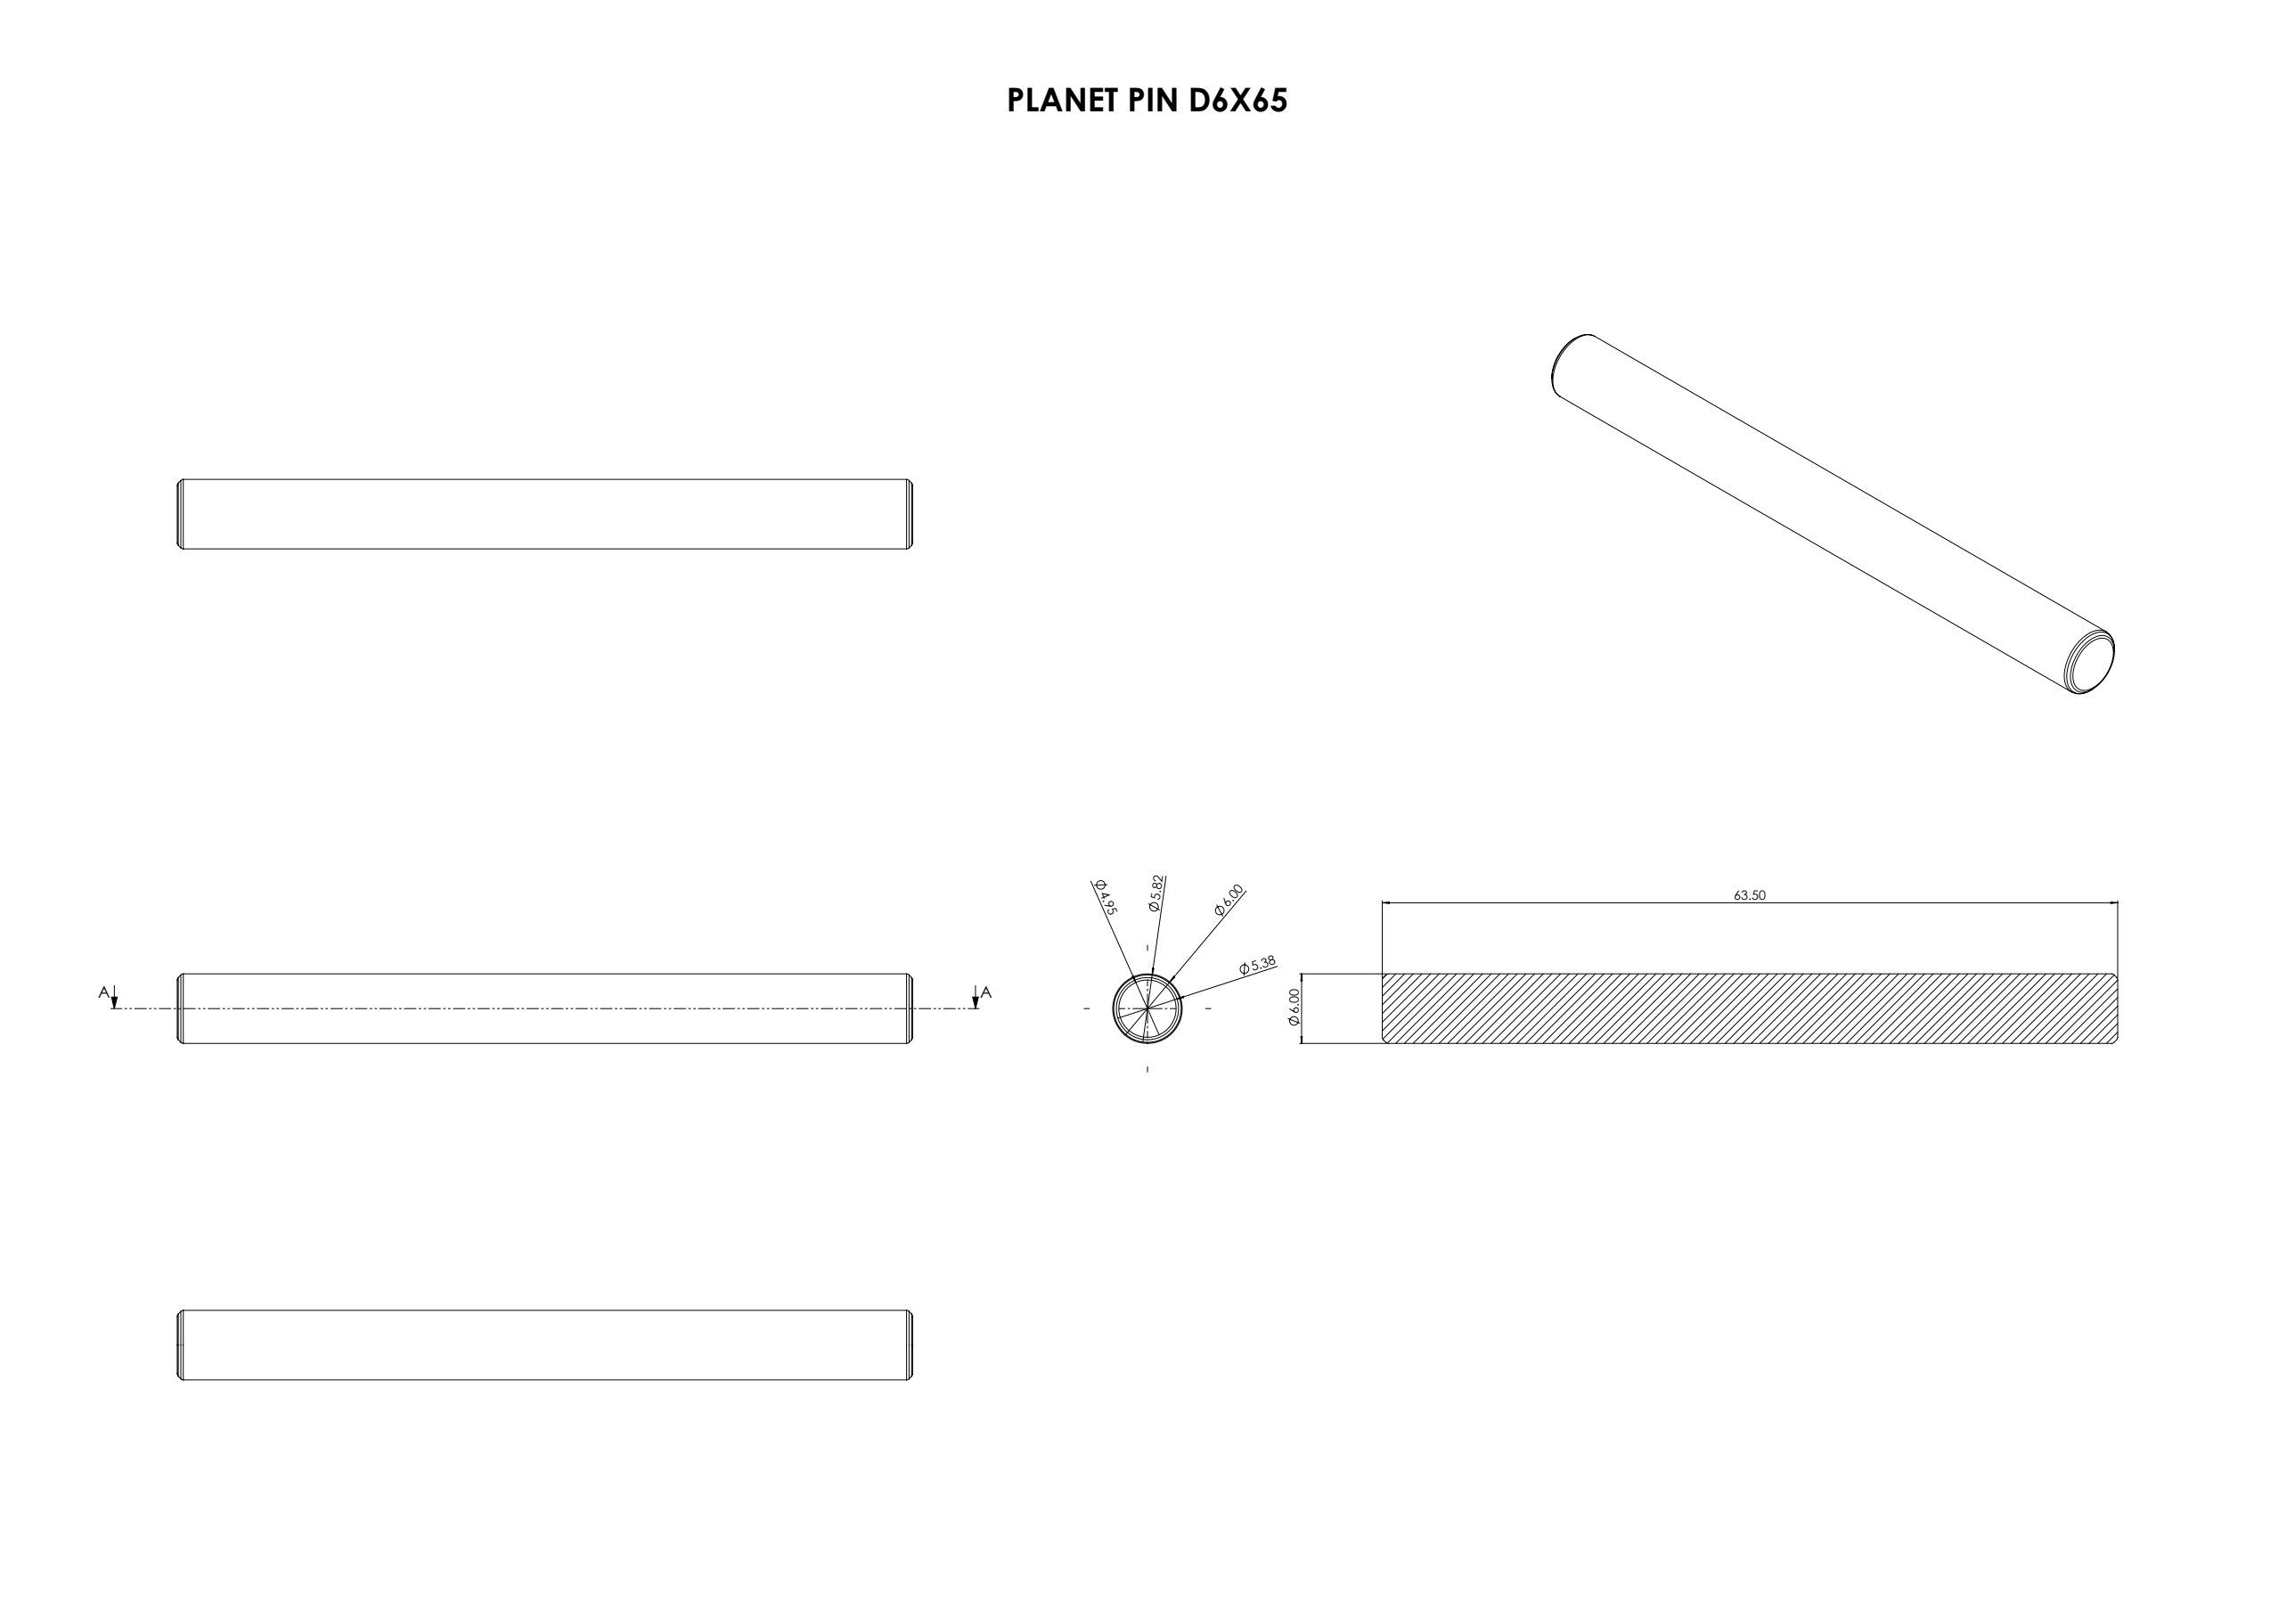
ISO-10303-21;
HEADER;
/* Generated by software containing ST-Developer
 * from STEP Tools, Inc. (www.steptools.com) 
 */

FILE_DESCRIPTION(
/* description */ (''),
/* implementation_level */ '2;1');

FILE_NAME(
/* name */ '04_Planet_Pin_D6x65.step',
/* time_stamp */ '2026-10-11T13:00:10-07:00',
/* author */ (''),
/* organization */ (''),
/* preprocessor_version */ 'ST-DEVELOPER v20.2',
/* originating_system */ 'Autodesk Translation Framework v15.15.0.0',
/* authorisation */ '');

FILE_SCHEMA (('AUTOMOTIVE_DESIGN { 1 0 10303 214 3 1 1 }'));
ENDSEC;

DATA;
#10=MECHANICAL_DESIGN_GEOMETRIC_PRESENTATION_REPRESENTATION('',(#361),#65563);
#145=TOROIDAL_SURFACE('',#21674,2.47573593128807,0.3);
#146=TOROIDAL_SURFACE('',#21683,2.7,0.3);
#147=TOROIDAL_SURFACE('',#21690,2.7,0.3);
#148=TOROIDAL_SURFACE('',#21697,2.47573593128807,0.3);
#339=SHAPE_REPRESENTATION_RELATIONSHIP('SRR','None',#65617,#350);
#350=ADVANCED_BREP_SHAPE_REPRESENTATION('',(#372),#65555);
#361=STYLED_ITEM('',(#65788),#372);
#372=MANIFOLD_SOLID_BREP('Body1',#20011);
#489=CONICAL_SURFACE('',#21679,2.8,0.785398163397448);
#490=CONICAL_SURFACE('',#21694,2.8,0.785398163397436);
#974=PLANE('',#21682);
#975=PLANE('',#21700);
#1978=FACE_OUTER_BOUND('',#3200,.T.);
#1979=FACE_OUTER_BOUND('',#3201,.T.);
#1980=FACE_OUTER_BOUND('',#3202,.T.);
#1981=FACE_OUTER_BOUND('',#3203,.T.);
#1982=FACE_OUTER_BOUND('',#3204,.T.);
#1983=FACE_OUTER_BOUND('',#3205,.T.);
#1984=FACE_OUTER_BOUND('',#3206,.T.);
#1985=FACE_OUTER_BOUND('',#3207,.T.);
#1986=FACE_OUTER_BOUND('',#3208,.T.);
#3200=EDGE_LOOP('',(#16702,#16703,#16704,#16705,#16706));
#3201=EDGE_LOOP('',(#16707,#16708,#16709,#16710,#16711,#16712));
#3202=EDGE_LOOP('',(#16713));
#3203=EDGE_LOOP('',(#16714,#16715,#16716,#16717,#16718,#16719));
#3204=EDGE_LOOP('',(#16720,#16721,#16722,#16723,#16724,#16725));
#3205=EDGE_LOOP('',(#16726,#16727,#16728,#16729,#16730,#16731));
#3206=EDGE_LOOP('',(#16732,#16733,#16734,#16735,#16736,#16737));
#3207=EDGE_LOOP('',(#16738,#16739,#16740,#16741,#16742));
#3208=EDGE_LOOP('',(#16743));
#4302=CIRCLE('',#21675,2.47573593128807);
#4303=CIRCLE('',#21676,0.3);
#4304=CIRCLE('',#21677,2.68786796564404);
#4305=CIRCLE('',#21678,2.68786796564404);
#4306=CIRCLE('',#21680,2.91213203435596);
#4307=CIRCLE('',#21681,2.91213203435596);
#4308=CIRCLE('',#21684,0.3);
#4309=CIRCLE('',#21685,3.);
#4310=CIRCLE('',#21686,3.);
#4311=CIRCLE('',#21688,3.);
#4312=CIRCLE('',#21689,3.);
#4313=CIRCLE('',#21691,0.3);
#4314=CIRCLE('',#21692,2.91213203435597);
#4315=CIRCLE('',#21693,2.91213203435597);
#4316=CIRCLE('',#21695,2.68786796564404);
#4317=CIRCLE('',#21696,2.68786796564404);
#4318=CIRCLE('',#21698,0.3);
#4319=CIRCLE('',#21699,2.47573593128807);
#6007=LINE('',#61837,#6899);
#6008=LINE('',#61850,#6900);
#6009=LINE('',#61862,#6901);
#6899=VECTOR('',#26046,2.8);
#6900=VECTOR('',#26063,3.);
#6901=VECTOR('',#26078,2.8);
#8647=VERTEX_POINT('',#61828);
#8648=VERTEX_POINT('',#61830);
#8649=VERTEX_POINT('',#61832);
#8650=VERTEX_POINT('',#61836);
#8651=VERTEX_POINT('',#61838);
#8652=VERTEX_POINT('',#61843);
#8653=VERTEX_POINT('',#61845);
#8654=VERTEX_POINT('',#61849);
#8655=VERTEX_POINT('',#61851);
#8656=VERTEX_POINT('',#61855);
#8657=VERTEX_POINT('',#61857);
#8658=VERTEX_POINT('',#61861);
#8659=VERTEX_POINT('',#61863);
#8660=VERTEX_POINT('',#61867);
#11384=EDGE_CURVE('',#8647,#8647,#4302,.T.);
#11385=EDGE_CURVE('',#8647,#8648,#4303,.T.);
#11386=EDGE_CURVE('',#8648,#8649,#4304,.T.);
#11387=EDGE_CURVE('',#8649,#8648,#4305,.T.);
#11388=EDGE_CURVE('',#8649,#8650,#6007,.T.);
#11389=EDGE_CURVE('',#8651,#8650,#4306,.T.);
#11390=EDGE_CURVE('',#8650,#8651,#4307,.T.);
#11391=EDGE_CURVE('',#8651,#8652,#4308,.T.);
#11392=EDGE_CURVE('',#8652,#8653,#4309,.T.);
#11393=EDGE_CURVE('',#8653,#8652,#4310,.T.);
#11394=EDGE_CURVE('',#8653,#8654,#6008,.T.);
#11395=EDGE_CURVE('',#8655,#8654,#4311,.T.);
#11396=EDGE_CURVE('',#8654,#8655,#4312,.T.);
#11397=EDGE_CURVE('',#8655,#8656,#4313,.T.);
#11398=EDGE_CURVE('',#8656,#8657,#4314,.T.);
#11399=EDGE_CURVE('',#8657,#8656,#4315,.T.);
#11400=EDGE_CURVE('',#8657,#8658,#6009,.T.);
#11401=EDGE_CURVE('',#8659,#8658,#4316,.T.);
#11402=EDGE_CURVE('',#8658,#8659,#4317,.T.);
#11403=EDGE_CURVE('',#8659,#8660,#4318,.T.);
#11404=EDGE_CURVE('',#8660,#8660,#4319,.T.);
#16702=ORIENTED_EDGE('',*,*,#11384,.T.);
#16703=ORIENTED_EDGE('',*,*,#11385,.T.);
#16704=ORIENTED_EDGE('',*,*,#11386,.T.);
#16705=ORIENTED_EDGE('',*,*,#11387,.T.);
#16706=ORIENTED_EDGE('',*,*,#11385,.F.);
#16707=ORIENTED_EDGE('',*,*,#11387,.F.);
#16708=ORIENTED_EDGE('',*,*,#11388,.T.);
#16709=ORIENTED_EDGE('',*,*,#11389,.F.);
#16710=ORIENTED_EDGE('',*,*,#11390,.F.);
#16711=ORIENTED_EDGE('',*,*,#11388,.F.);
#16712=ORIENTED_EDGE('',*,*,#11386,.F.);
#16713=ORIENTED_EDGE('',*,*,#11384,.F.);
#16714=ORIENTED_EDGE('',*,*,#11389,.T.);
#16715=ORIENTED_EDGE('',*,*,#11390,.T.);
#16716=ORIENTED_EDGE('',*,*,#11391,.T.);
#16717=ORIENTED_EDGE('',*,*,#11392,.T.);
#16718=ORIENTED_EDGE('',*,*,#11393,.T.);
#16719=ORIENTED_EDGE('',*,*,#11391,.F.);
#16720=ORIENTED_EDGE('',*,*,#11393,.F.);
#16721=ORIENTED_EDGE('',*,*,#11394,.T.);
#16722=ORIENTED_EDGE('',*,*,#11395,.F.);
#16723=ORIENTED_EDGE('',*,*,#11396,.F.);
#16724=ORIENTED_EDGE('',*,*,#11394,.F.);
#16725=ORIENTED_EDGE('',*,*,#11392,.F.);
#16726=ORIENTED_EDGE('',*,*,#11395,.T.);
#16727=ORIENTED_EDGE('',*,*,#11396,.T.);
#16728=ORIENTED_EDGE('',*,*,#11397,.T.);
#16729=ORIENTED_EDGE('',*,*,#11398,.T.);
#16730=ORIENTED_EDGE('',*,*,#11399,.T.);
#16731=ORIENTED_EDGE('',*,*,#11397,.F.);
#16732=ORIENTED_EDGE('',*,*,#11399,.F.);
#16733=ORIENTED_EDGE('',*,*,#11400,.T.);
#16734=ORIENTED_EDGE('',*,*,#11401,.F.);
#16735=ORIENTED_EDGE('',*,*,#11402,.F.);
#16736=ORIENTED_EDGE('',*,*,#11400,.F.);
#16737=ORIENTED_EDGE('',*,*,#11398,.F.);
#16738=ORIENTED_EDGE('',*,*,#11401,.T.);
#16739=ORIENTED_EDGE('',*,*,#11402,.T.);
#16740=ORIENTED_EDGE('',*,*,#11403,.T.);
#16741=ORIENTED_EDGE('',*,*,#11404,.T.);
#16742=ORIENTED_EDGE('',*,*,#11403,.F.);
#16743=ORIENTED_EDGE('',*,*,#11404,.F.);
#18716=CYLINDRICAL_SURFACE('',#21687,3.);
#19674=ADVANCED_FACE('',(#1978),#145,.T.);
#19675=ADVANCED_FACE('',(#1979),#489,.T.);
#19676=ADVANCED_FACE('',(#1980),#974,.T.);
#19677=ADVANCED_FACE('',(#1981),#146,.T.);
#19678=ADVANCED_FACE('',(#1982),#18716,.T.);
#19679=ADVANCED_FACE('',(#1983),#147,.T.);
#19680=ADVANCED_FACE('',(#1984),#490,.T.);
#19681=ADVANCED_FACE('',(#1985),#148,.T.);
#19682=ADVANCED_FACE('',(#1986),#975,.T.);
#20011=CLOSED_SHELL('',(#19674,#19675,#19676,#19677,#19678,#19679,#19680,
#19681,#19682));
#21673=AXIS2_PLACEMENT_3D('',#61826,#26032,#26033);
#21674=AXIS2_PLACEMENT_3D('',#61827,#26034,#26035);
#21675=AXIS2_PLACEMENT_3D('',#61829,#26036,#26037);
#21676=AXIS2_PLACEMENT_3D('',#61831,#26038,#26039);
#21677=AXIS2_PLACEMENT_3D('',#61833,#26040,#26041);
#21678=AXIS2_PLACEMENT_3D('',#61834,#26042,#26043);
#21679=AXIS2_PLACEMENT_3D('',#61835,#26044,#26045);
#21680=AXIS2_PLACEMENT_3D('',#61839,#26047,#26048);
#21681=AXIS2_PLACEMENT_3D('',#61840,#26049,#26050);
#21682=AXIS2_PLACEMENT_3D('',#61841,#26051,#26052);
#21683=AXIS2_PLACEMENT_3D('',#61842,#26053,#26054);
#21684=AXIS2_PLACEMENT_3D('',#61844,#26055,#26056);
#21685=AXIS2_PLACEMENT_3D('',#61846,#26057,#26058);
#21686=AXIS2_PLACEMENT_3D('',#61847,#26059,#26060);
#21687=AXIS2_PLACEMENT_3D('',#61848,#26061,#26062);
#21688=AXIS2_PLACEMENT_3D('',#61852,#26064,#26065);
#21689=AXIS2_PLACEMENT_3D('',#61853,#26066,#26067);
#21690=AXIS2_PLACEMENT_3D('',#61854,#26068,#26069);
#21691=AXIS2_PLACEMENT_3D('',#61856,#26070,#26071);
#21692=AXIS2_PLACEMENT_3D('',#61858,#26072,#26073);
#21693=AXIS2_PLACEMENT_3D('',#61859,#26074,#26075);
#21694=AXIS2_PLACEMENT_3D('',#61860,#26076,#26077);
#21695=AXIS2_PLACEMENT_3D('',#61864,#26079,#26080);
#21696=AXIS2_PLACEMENT_3D('',#61865,#26081,#26082);
#21697=AXIS2_PLACEMENT_3D('',#61866,#26083,#26084);
#21698=AXIS2_PLACEMENT_3D('',#61868,#26085,#26086);
#21699=AXIS2_PLACEMENT_3D('',#61869,#26087,#26088);
#21700=AXIS2_PLACEMENT_3D('',#61870,#26089,#26090);
#26032=DIRECTION('axis',(0.,0.,1.));
#26033=DIRECTION('refdir',(1.,0.,0.));
#26034=DIRECTION('center_axis',(1.,0.,0.));
#26035=DIRECTION('ref_axis',(0.,0.,-1.));
#26036=DIRECTION('center_axis',(-1.,0.,0.));
#26037=DIRECTION('ref_axis',(0.,-1.,1.83697019872103E-16));
#26038=DIRECTION('center_axis',(0.,-1.,-1.22464679914735E-16));
#26039=DIRECTION('ref_axis',(0.,-1.22464679914735E-16,1.));
#26040=DIRECTION('center_axis',(1.,0.,0.));
#26041=DIRECTION('ref_axis',(0.,-1.,3.06161699786838E-17));
#26042=DIRECTION('center_axis',(1.,0.,0.));
#26043=DIRECTION('ref_axis',(0.,-1.,3.06161699786838E-17));
#26044=DIRECTION('center_axis',(-1.,0.,0.));
#26045=DIRECTION('ref_axis',(0.,1.,0.));
#26046=DIRECTION('',(-0.707106781186548,-0.707106781186547,-8.65956056235493E-17));
#26047=DIRECTION('center_axis',(-1.,0.,0.));
#26048=DIRECTION('ref_axis',(0.,-1.,3.06161699786838E-17));
#26049=DIRECTION('center_axis',(-1.,0.,0.));
#26050=DIRECTION('ref_axis',(0.,-1.,3.06161699786838E-17));
#26051=DIRECTION('center_axis',(1.,0.,0.));
#26052=DIRECTION('ref_axis',(0.,0.,-1.));
#26053=DIRECTION('center_axis',(1.,0.,0.));
#26054=DIRECTION('ref_axis',(0.,0.,-1.));
#26055=DIRECTION('center_axis',(0.,-1.,-1.22464679914735E-16));
#26056=DIRECTION('ref_axis',(0.,-1.22464679914735E-16,1.));
#26057=DIRECTION('center_axis',(1.,0.,0.));
#26058=DIRECTION('ref_axis',(0.,-1.,1.83697019872103E-16));
#26059=DIRECTION('center_axis',(1.,0.,0.));
#26060=DIRECTION('ref_axis',(0.,-1.,1.83697019872103E-16));
#26061=DIRECTION('center_axis',(1.,0.,0.));
#26062=DIRECTION('ref_axis',(0.,1.,0.));
#26063=DIRECTION('',(-1.,0.,0.));
#26064=DIRECTION('center_axis',(-1.,0.,0.));
#26065=DIRECTION('ref_axis',(0.,-1.,1.83697019872103E-16));
#26066=DIRECTION('center_axis',(-1.,0.,0.));
#26067=DIRECTION('ref_axis',(0.,-1.,1.83697019872103E-16));
#26068=DIRECTION('center_axis',(1.,0.,0.));
#26069=DIRECTION('ref_axis',(0.,0.,-1.));
#26070=DIRECTION('center_axis',(0.,-1.,-1.22464679914735E-16));
#26071=DIRECTION('ref_axis',(0.,-1.22464679914735E-16,1.));
#26072=DIRECTION('center_axis',(1.,0.,0.));
#26073=DIRECTION('ref_axis',(0.,-1.,3.06161699786838E-17));
#26074=DIRECTION('center_axis',(1.,0.,0.));
#26075=DIRECTION('ref_axis',(0.,-1.,3.06161699786838E-17));
#26076=DIRECTION('center_axis',(1.,0.,0.));
#26077=DIRECTION('ref_axis',(0.,1.,0.));
#26078=DIRECTION('',(-0.707106781186556,0.707106781186539,8.65956056235483E-17));
#26079=DIRECTION('center_axis',(-1.,0.,0.));
#26080=DIRECTION('ref_axis',(0.,-1.,3.06161699786838E-17));
#26081=DIRECTION('center_axis',(-1.,0.,0.));
#26082=DIRECTION('ref_axis',(0.,-1.,3.06161699786838E-17));
#26083=DIRECTION('center_axis',(1.,0.,0.));
#26084=DIRECTION('ref_axis',(0.,0.,-1.));
#26085=DIRECTION('center_axis',(0.,-1.,-1.22464679914735E-16));
#26086=DIRECTION('ref_axis',(0.,-1.22464679914735E-16,1.));
#26087=DIRECTION('center_axis',(1.,0.,0.));
#26088=DIRECTION('ref_axis',(0.,-1.,1.83697019872103E-16));
#26089=DIRECTION('center_axis',(-1.,0.,0.));
#26090=DIRECTION('ref_axis',(0.,0.,1.));
#61826=CARTESIAN_POINT('',(0.,0.,0.));
#61827=CARTESIAN_POINT('Origin',(-15.8,0.,0.));
#61828=CARTESIAN_POINT('',(-15.5,-3.03190208378603E-16,2.47573593128807));
#61829=CARTESIAN_POINT('Origin',(-15.5,0.,0.));
#61830=CARTESIAN_POINT('',(-15.587867965644,-3.29168890065668E-16,2.68786796564404));
#61831=CARTESIAN_POINT('Origin',(-15.8,-3.03190208378603E-16,2.47573593128807));
#61832=CARTESIAN_POINT('',(-15.587867965644,-2.68786796564404,-3.29168890065668E-16));
#61833=CARTESIAN_POINT('Origin',(-15.587867965644,0.,-4.11461112582085E-16));
#61834=CARTESIAN_POINT('Origin',(-15.587867965644,0.,-4.11461112582085E-16));
#61835=CARTESIAN_POINT('Origin',(-15.7,0.,0.));
#61836=CARTESIAN_POINT('',(-15.812132034356,-2.91213203435596,-3.5663331745685E-16));
#61837=CARTESIAN_POINT('',(-15.7,-2.8,-3.42901103761259E-16));
#61838=CARTESIAN_POINT('',(-15.812132034356,-3.5663331745685E-16,2.91213203435596));
#61839=CARTESIAN_POINT('Origin',(-15.812132034356,0.,-4.45791646821063E-16));
#61840=CARTESIAN_POINT('Origin',(-15.812132034356,0.,-4.45791646821063E-16));
#61841=CARTESIAN_POINT('Origin',(-15.5,0.,0.));
#61842=CARTESIAN_POINT('Origin',(-16.0242640687119,0.,0.));
#61843=CARTESIAN_POINT('',(-16.0242640687119,-3.67394039744206E-16,3.));
#61844=CARTESIAN_POINT('Origin',(-16.0242640687119,-3.30654635769785E-16,
2.7));
#61845=CARTESIAN_POINT('',(-16.0242640687119,-3.,-3.67394039744206E-16));
#61846=CARTESIAN_POINT('Origin',(-16.0242640687119,0.,0.));
#61847=CARTESIAN_POINT('Origin',(-16.0242640687119,0.,0.));
#61848=CARTESIAN_POINT('Origin',(-47.25,0.,0.));
#61849=CARTESIAN_POINT('',(-78.4757359312881,-3.,-3.67394039744206E-16));
#61850=CARTESIAN_POINT('',(-47.25,-3.,-3.67394039744206E-16));
#61851=CARTESIAN_POINT('',(-78.4757359312881,-3.67394039744206E-16,3.));
#61852=CARTESIAN_POINT('Origin',(-78.4757359312881,0.,0.));
#61853=CARTESIAN_POINT('Origin',(-78.4757359312881,0.,0.));
#61854=CARTESIAN_POINT('Origin',(-78.4757359312881,0.,0.));
#61855=CARTESIAN_POINT('',(-78.687867965644,-3.5663331745685E-16,2.91213203435596));
#61856=CARTESIAN_POINT('Origin',(-78.4757359312881,-3.30654635769785E-16,
2.7));
#61857=CARTESIAN_POINT('',(-78.687867965644,-2.91213203435597,-3.5663331745685E-16));
#61858=CARTESIAN_POINT('Origin',(-78.687867965644,0.,-4.45791646821063E-16));
#61859=CARTESIAN_POINT('Origin',(-78.687867965644,0.,-4.45791646821063E-16));
#61860=CARTESIAN_POINT('Origin',(-78.8,0.,0.));
#61861=CARTESIAN_POINT('',(-78.912132034356,-2.68786796564404,-3.29168890065668E-16));
#61862=CARTESIAN_POINT('',(-78.8,-2.8,-3.42901103761259E-16));
#61863=CARTESIAN_POINT('',(-78.912132034356,-3.29168890065668E-16,2.68786796564404));
#61864=CARTESIAN_POINT('Origin',(-78.912132034356,0.,-4.11461112582085E-16));
#61865=CARTESIAN_POINT('Origin',(-78.912132034356,0.,-4.11461112582085E-16));
#61866=CARTESIAN_POINT('Origin',(-78.7,0.,0.));
#61867=CARTESIAN_POINT('',(-79.,-3.03190208378603E-16,2.47573593128807));
#61868=CARTESIAN_POINT('Origin',(-78.7,-3.03190208378603E-16,2.47573593128807));
#61869=CARTESIAN_POINT('Origin',(-79.,0.,0.));
#61870=CARTESIAN_POINT('Origin',(-79.,2.6,0.));
#65542=UNCERTAINTY_MEASURE_WITH_UNIT(LENGTH_MEASURE(0.01),#65564,
'DISTANCE_ACCURACY_VALUE',
'Maximum model space distance between geometric entities at asserted c
onnectivities');
#65550=UNCERTAINTY_MEASURE_WITH_UNIT(LENGTH_MEASURE(0.01),#65564,
'DISTANCE_ACCURACY_VALUE',
'Maximum model space distance between geometric entities at asserted c
onnectivities');
#65555=(
GEOMETRIC_REPRESENTATION_CONTEXT(3)
GLOBAL_UNCERTAINTY_ASSIGNED_CONTEXT((#65542))
GLOBAL_UNIT_ASSIGNED_CONTEXT((#65564,#65566,#65567))
REPRESENTATION_CONTEXT('','3D')
);
#65563=(
GEOMETRIC_REPRESENTATION_CONTEXT(3)
GLOBAL_UNCERTAINTY_ASSIGNED_CONTEXT((#65550))
GLOBAL_UNIT_ASSIGNED_CONTEXT((#65564,#65566,#65567))
REPRESENTATION_CONTEXT('','3D')
);
#65564=(
LENGTH_UNIT()
NAMED_UNIT(*)
SI_UNIT(.MILLI.,.METRE.)
);
#65566=(
NAMED_UNIT(*)
PLANE_ANGLE_UNIT()
SI_UNIT($,.RADIAN.)
);
#65567=(
NAMED_UNIT(*)
SI_UNIT($,.STERADIAN.)
SOLID_ANGLE_UNIT()
);
#65572=SHAPE_DEFINITION_REPRESENTATION(#65584,#65617);
#65584=PRODUCT_DEFINITION_SHAPE('',$,#65630);
#65617=SHAPE_REPRESENTATION('',(#21673),#65555);
#65625=PRODUCT_DEFINITION_CONTEXT('part definition',#65663,'design');
#65630=PRODUCT_DEFINITION('2026-10-10-05-45-27-457',
'04_Planet_Pin_D6x65',#65642,#65625);
#65642=PRODUCT_DEFINITION_FORMATION('',$,#65669);
#65663=APPLICATION_CONTEXT(
'Core Data for Automotive Mechanical Design Process');
#65664=PRODUCT_CONTEXT('part definition',#65663,'mechanical');
#65669=PRODUCT('2026-10-10-05-45-27-457','04_Planet_Pin_D6x65',$,(#65664));
#65782=COLOUR_RGB('Grey',0.48,0.52,0.57);
#65783=FILL_AREA_STYLE_COLOUR('',#65782);
#65784=FILL_AREA_STYLE('',(#65783));
#65785=SURFACE_STYLE_FILL_AREA(#65784);
#65786=SURFACE_SIDE_STYLE('',(#65785));
#65787=SURFACE_STYLE_USAGE(.BOTH.,#65786);
#65788=PRESENTATION_STYLE_ASSIGNMENT((#65787));
ENDSEC;
END-ISO-10303-21;
